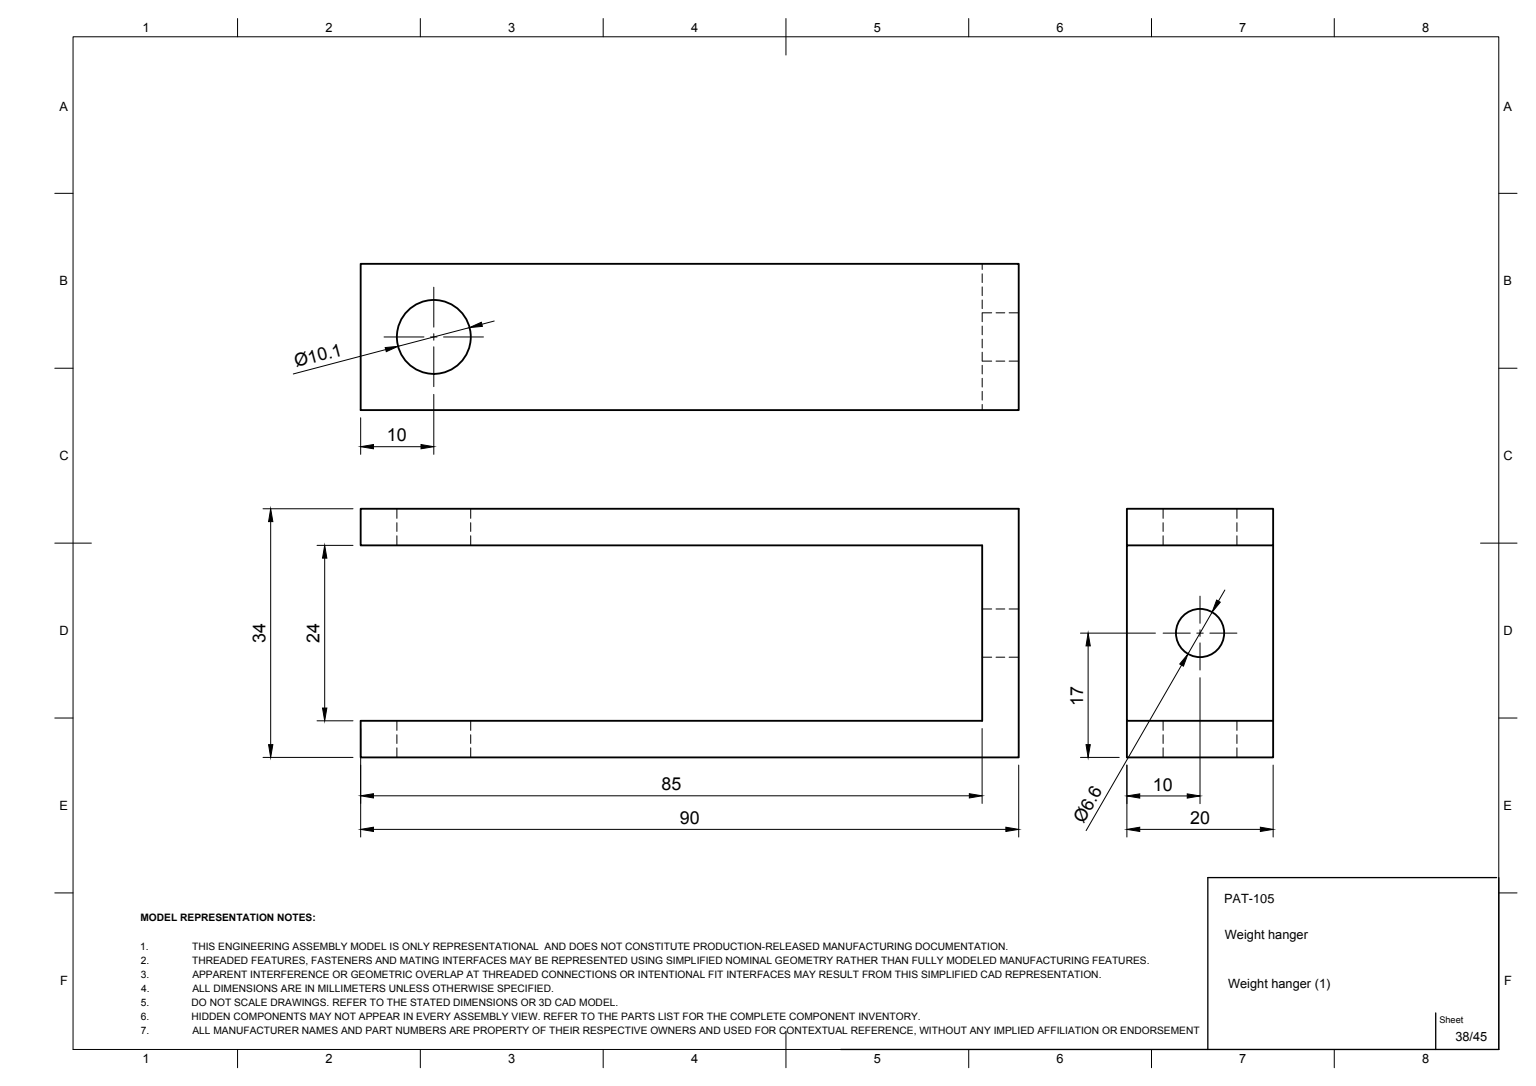
ISO-10303-21;
HEADER;
/* Generated by software containing ST-Developer
 * from STEP Tools, Inc. (www.steptools.com) 
 */

FILE_DESCRIPTION(
/* description */ ('Torque wrench calibration arm'),
/* implementation_level */ '2;1');

FILE_NAME(
/* name */ 'Weight hanger.step',
/* time_stamp */ '2026-10-28T03:24:52-07:00',
/* author */ (''),
/* organization */ (''),
/* preprocessor_version */ 'ST-DEVELOPER v20.2',
/* originating_system */ 'Autodesk Translation Framework v15.17.0.0',
/* authorisation */ '');

FILE_SCHEMA (('AUTOMOTIVE_DESIGN { 1 0 10303 214 3 1 1 }'));
ENDSEC;

DATA;
#10=MECHANICAL_DESIGN_GEOMETRIC_PRESENTATION_REPRESENTATION('',(#471),#12783);
#380=SHAPE_REPRESENTATION_RELATIONSHIP('SRR','None',#12965,#417);
#417=ADVANCED_BREP_SHAPE_REPRESENTATION('',(#523),#12774);
#471=STYLED_ITEM('',(#13198),#523);
#523=MANIFOLD_SOLID_BREP('Body1',#6542);
#631=FACE_BOUND('',#1709,.T.);
#632=FACE_BOUND('',#1712,.T.);
#633=FACE_BOUND('',#1714,.T.);
#634=FACE_BOUND('',#1716,.T.);
#635=FACE_BOUND('',#1719,.T.);
#636=FACE_BOUND('',#1723,.T.);
#838=PLANE('',#7695);
#839=PLANE('',#7696);
#840=PLANE('',#7697);
#841=PLANE('',#7698);
#842=PLANE('',#7699);
#843=PLANE('',#7700);
#844=PLANE('',#7701);
#845=PLANE('',#7702);
#846=PLANE('',#7703);
#847=PLANE('',#7704);
#1210=FACE_OUTER_BOUND('',#1705,.T.);
#1211=FACE_OUTER_BOUND('',#1706,.T.);
#1212=FACE_OUTER_BOUND('',#1707,.T.);
#1213=FACE_OUTER_BOUND('',#1708,.T.);
#1214=FACE_OUTER_BOUND('',#1710,.T.);
#1215=FACE_OUTER_BOUND('',#1711,.T.);
#1216=FACE_OUTER_BOUND('',#1713,.T.);
#1217=FACE_OUTER_BOUND('',#1715,.T.);
#1218=FACE_OUTER_BOUND('',#1717,.T.);
#1219=FACE_OUTER_BOUND('',#1718,.T.);
#1220=FACE_OUTER_BOUND('',#1720,.T.);
#1221=FACE_OUTER_BOUND('',#1721,.T.);
#1222=FACE_OUTER_BOUND('',#1722,.T.);
#1705=EDGE_LOOP('',(#5771,#5772,#5773,#5774));
#1706=EDGE_LOOP('',(#5775,#5776,#5777,#5778));
#1707=EDGE_LOOP('',(#5779,#5780,#5781,#5782));
#1708=EDGE_LOOP('',(#5783,#5784,#5785,#5786));
#1709=EDGE_LOOP('',(#5787));
#1710=EDGE_LOOP('',(#5788,#5789,#5790,#5791));
#1711=EDGE_LOOP('',(#5792,#5793,#5794,#5795));
#1712=EDGE_LOOP('',(#5796));
#1713=EDGE_LOOP('',(#5797,#5798,#5799,#5800));
#1714=EDGE_LOOP('',(#5801));
#1715=EDGE_LOOP('',(#5802,#5803,#5804,#5805));
#1716=EDGE_LOOP('',(#5806));
#1717=EDGE_LOOP('',(#5807,#5808,#5809,#5810,#5811,#5812,#5813,#5814));
#1718=EDGE_LOOP('',(#5815,#5816,#5817,#5818));
#1719=EDGE_LOOP('',(#5819));
#1720=EDGE_LOOP('',(#5820,#5821,#5822,#5823,#5824,#5825,#5826,#5827));
#1721=EDGE_LOOP('',(#5828,#5829,#5830,#5831));
#1722=EDGE_LOOP('',(#5832,#5833,#5834,#5835));
#1723=EDGE_LOOP('',(#5836));
#2136=LINE('',#12440,#2551);
#2137=LINE('',#12446,#2552);
#2138=LINE('',#12452,#2553);
#2139=LINE('',#12457,#2554);
#2140=LINE('',#12459,#2555);
#2141=LINE('',#12461,#2556);
#2142=LINE('',#12462,#2557);
#2143=LINE('',#12466,#2558);
#2144=LINE('',#12468,#2559);
#2145=LINE('',#12470,#2560);
#2146=LINE('',#12471,#2561);
#2147=LINE('',#12474,#2562);
#2148=LINE('',#12476,#2563);
#2149=LINE('',#12477,#2564);
#2150=LINE('',#12479,#2565);
#2151=LINE('',#12480,#2566);
#2152=LINE('',#12483,#2567);
#2153=LINE('',#12485,#2568);
#2154=LINE('',#12486,#2569);
#2155=LINE('',#12490,#2570);
#2156=LINE('',#12491,#2571);
#2157=LINE('',#12492,#2572);
#2158=LINE('',#12495,#2573);
#2159=LINE('',#12496,#2574);
#2160=LINE('',#12499,#2575);
#2161=LINE('',#12500,#2576);
#2162=LINE('',#12502,#2577);
#2551=VECTOR('',#9616,0.329999999999998);
#2552=VECTOR('',#9623,0.505000000000003);
#2553=VECTOR('',#9630,0.505000000000003);
#2554=VECTOR('',#9635,1.);
#2555=VECTOR('',#9636,1.);
#2556=VECTOR('',#9637,1.);
#2557=VECTOR('',#9638,1.);
#2558=VECTOR('',#9641,1.);
#2559=VECTOR('',#9642,1.);
#2560=VECTOR('',#9643,1.);
#2561=VECTOR('',#9644,1.);
#2562=VECTOR('',#9647,1.);
#2563=VECTOR('',#9648,1.);
#2564=VECTOR('',#9649,1.);
#2565=VECTOR('',#9652,1.);
#2566=VECTOR('',#9653,1.);
#2567=VECTOR('',#9656,1.);
#2568=VECTOR('',#9657,1.);
#2569=VECTOR('',#9658,1.);
#2570=VECTOR('',#9661,1.);
#2571=VECTOR('',#9662,1.);
#2572=VECTOR('',#9663,1.);
#2573=VECTOR('',#9666,1.);
#2574=VECTOR('',#9667,1.);
#2575=VECTOR('',#9670,1.);
#2576=VECTOR('',#9671,1.);
#2577=VECTOR('',#9674,1.);
#2928=CIRCLE('',#7687,0.329999999999998);
#2929=CIRCLE('',#7688,0.329999999999998);
#2930=CIRCLE('',#7690,0.505000000000003);
#2931=CIRCLE('',#7691,0.505000000000003);
#2932=CIRCLE('',#7693,0.505000000000003);
#2933=CIRCLE('',#7694,0.505000000000003);
#3462=VERTEX_POINT('',#12437);
#3463=VERTEX_POINT('',#12439);
#3464=VERTEX_POINT('',#12443);
#3465=VERTEX_POINT('',#12445);
#3466=VERTEX_POINT('',#12449);
#3467=VERTEX_POINT('',#12451);
#3468=VERTEX_POINT('',#12455);
#3469=VERTEX_POINT('',#12456);
#3470=VERTEX_POINT('',#12458);
#3471=VERTEX_POINT('',#12460);
#3472=VERTEX_POINT('',#12464);
#3473=VERTEX_POINT('',#12465);
#3474=VERTEX_POINT('',#12467);
#3475=VERTEX_POINT('',#12469);
#3476=VERTEX_POINT('',#12473);
#3477=VERTEX_POINT('',#12475);
#3478=VERTEX_POINT('',#12482);
#3479=VERTEX_POINT('',#12484);
#3480=VERTEX_POINT('',#12488);
#3481=VERTEX_POINT('',#12489);
#3482=VERTEX_POINT('',#12494);
#3483=VERTEX_POINT('',#12498);
#4243=EDGE_CURVE('',#3462,#3462,#2928,.T.);
#4244=EDGE_CURVE('',#3462,#3463,#2136,.T.);
#4245=EDGE_CURVE('',#3463,#3463,#2929,.T.);
#4246=EDGE_CURVE('',#3464,#3464,#2930,.T.);
#4247=EDGE_CURVE('',#3464,#3465,#2137,.T.);
#4248=EDGE_CURVE('',#3465,#3465,#2931,.T.);
#4249=EDGE_CURVE('',#3466,#3466,#2932,.T.);
#4250=EDGE_CURVE('',#3466,#3467,#2138,.T.);
#4251=EDGE_CURVE('',#3467,#3467,#2933,.T.);
#4252=EDGE_CURVE('',#3468,#3469,#2139,.T.);
#4253=EDGE_CURVE('',#3468,#3470,#2140,.T.);
#4254=EDGE_CURVE('',#3471,#3470,#2141,.T.);
#4255=EDGE_CURVE('',#3469,#3471,#2142,.T.);
#4256=EDGE_CURVE('',#3472,#3473,#2143,.T.);
#4257=EDGE_CURVE('',#3472,#3474,#2144,.T.);
#4258=EDGE_CURVE('',#3475,#3474,#2145,.T.);
#4259=EDGE_CURVE('',#3473,#3475,#2146,.T.);
#4260=EDGE_CURVE('',#3474,#3476,#2147,.T.);
#4261=EDGE_CURVE('',#3476,#3477,#2148,.T.);
#4262=EDGE_CURVE('',#3477,#3475,#2149,.T.);
#4263=EDGE_CURVE('',#3470,#3472,#2150,.T.);
#4264=EDGE_CURVE('',#3473,#3471,#2151,.T.);
#4265=EDGE_CURVE('',#3469,#3478,#2152,.T.);
#4266=EDGE_CURVE('',#3478,#3479,#2153,.T.);
#4267=EDGE_CURVE('',#3479,#3468,#2154,.T.);
#4268=EDGE_CURVE('',#3480,#3481,#2155,.T.);
#4269=EDGE_CURVE('',#3480,#3478,#2156,.T.);
#4270=EDGE_CURVE('',#3481,#3477,#2157,.T.);
#4271=EDGE_CURVE('',#3481,#3482,#2158,.T.);
#4272=EDGE_CURVE('',#3482,#3476,#2159,.T.);
#4273=EDGE_CURVE('',#3482,#3483,#2160,.T.);
#4274=EDGE_CURVE('',#3483,#3479,#2161,.T.);
#4275=EDGE_CURVE('',#3483,#3480,#2162,.T.);
#5771=ORIENTED_EDGE('',*,*,#4243,.F.);
#5772=ORIENTED_EDGE('',*,*,#4244,.T.);
#5773=ORIENTED_EDGE('',*,*,#4245,.F.);
#5774=ORIENTED_EDGE('',*,*,#4244,.F.);
#5775=ORIENTED_EDGE('',*,*,#4246,.F.);
#5776=ORIENTED_EDGE('',*,*,#4247,.T.);
#5777=ORIENTED_EDGE('',*,*,#4248,.F.);
#5778=ORIENTED_EDGE('',*,*,#4247,.F.);
#5779=ORIENTED_EDGE('',*,*,#4249,.F.);
#5780=ORIENTED_EDGE('',*,*,#4250,.T.);
#5781=ORIENTED_EDGE('',*,*,#4251,.F.);
#5782=ORIENTED_EDGE('',*,*,#4250,.F.);
#5783=ORIENTED_EDGE('',*,*,#4252,.F.);
#5784=ORIENTED_EDGE('',*,*,#4253,.T.);
#5785=ORIENTED_EDGE('',*,*,#4254,.F.);
#5786=ORIENTED_EDGE('',*,*,#4255,.F.);
#5787=ORIENTED_EDGE('',*,*,#4245,.T.);
#5788=ORIENTED_EDGE('',*,*,#4256,.F.);
#5789=ORIENTED_EDGE('',*,*,#4257,.T.);
#5790=ORIENTED_EDGE('',*,*,#4258,.F.);
#5791=ORIENTED_EDGE('',*,*,#4259,.F.);
#5792=ORIENTED_EDGE('',*,*,#4258,.T.);
#5793=ORIENTED_EDGE('',*,*,#4260,.T.);
#5794=ORIENTED_EDGE('',*,*,#4261,.T.);
#5795=ORIENTED_EDGE('',*,*,#4262,.T.);
#5796=ORIENTED_EDGE('',*,*,#4251,.T.);
#5797=ORIENTED_EDGE('',*,*,#4254,.T.);
#5798=ORIENTED_EDGE('',*,*,#4263,.T.);
#5799=ORIENTED_EDGE('',*,*,#4256,.T.);
#5800=ORIENTED_EDGE('',*,*,#4264,.T.);
#5801=ORIENTED_EDGE('',*,*,#4249,.T.);
#5802=ORIENTED_EDGE('',*,*,#4252,.T.);
#5803=ORIENTED_EDGE('',*,*,#4265,.T.);
#5804=ORIENTED_EDGE('',*,*,#4266,.T.);
#5805=ORIENTED_EDGE('',*,*,#4267,.T.);
#5806=ORIENTED_EDGE('',*,*,#4248,.T.);
#5807=ORIENTED_EDGE('',*,*,#4268,.F.);
#5808=ORIENTED_EDGE('',*,*,#4269,.T.);
#5809=ORIENTED_EDGE('',*,*,#4265,.F.);
#5810=ORIENTED_EDGE('',*,*,#4255,.T.);
#5811=ORIENTED_EDGE('',*,*,#4264,.F.);
#5812=ORIENTED_EDGE('',*,*,#4259,.T.);
#5813=ORIENTED_EDGE('',*,*,#4262,.F.);
#5814=ORIENTED_EDGE('',*,*,#4270,.F.);
#5815=ORIENTED_EDGE('',*,*,#4271,.F.);
#5816=ORIENTED_EDGE('',*,*,#4270,.T.);
#5817=ORIENTED_EDGE('',*,*,#4261,.F.);
#5818=ORIENTED_EDGE('',*,*,#4272,.F.);
#5819=ORIENTED_EDGE('',*,*,#4243,.T.);
#5820=ORIENTED_EDGE('',*,*,#4273,.F.);
#5821=ORIENTED_EDGE('',*,*,#4272,.T.);
#5822=ORIENTED_EDGE('',*,*,#4260,.F.);
#5823=ORIENTED_EDGE('',*,*,#4257,.F.);
#5824=ORIENTED_EDGE('',*,*,#4263,.F.);
#5825=ORIENTED_EDGE('',*,*,#4253,.F.);
#5826=ORIENTED_EDGE('',*,*,#4267,.F.);
#5827=ORIENTED_EDGE('',*,*,#4274,.F.);
#5828=ORIENTED_EDGE('',*,*,#4275,.F.);
#5829=ORIENTED_EDGE('',*,*,#4274,.T.);
#5830=ORIENTED_EDGE('',*,*,#4266,.F.);
#5831=ORIENTED_EDGE('',*,*,#4269,.F.);
#5832=ORIENTED_EDGE('',*,*,#4275,.T.);
#5833=ORIENTED_EDGE('',*,*,#4268,.T.);
#5834=ORIENTED_EDGE('',*,*,#4271,.T.);
#5835=ORIENTED_EDGE('',*,*,#4273,.T.);
#5836=ORIENTED_EDGE('',*,*,#4246,.T.);
#6080=CYLINDRICAL_SURFACE('',#7686,0.329999999999998);
#6081=CYLINDRICAL_SURFACE('',#7689,0.505000000000003);
#6082=CYLINDRICAL_SURFACE('',#7692,0.505000000000003);
#6435=ADVANCED_FACE('',(#1210),#6080,.F.);
#6436=ADVANCED_FACE('',(#1211),#6081,.F.);
#6437=ADVANCED_FACE('',(#1212),#6082,.F.);
#6438=ADVANCED_FACE('',(#1213,#631),#838,.T.);
#6439=ADVANCED_FACE('',(#1214),#839,.T.);
#6440=ADVANCED_FACE('',(#1215,#632),#840,.T.);
#6441=ADVANCED_FACE('',(#1216,#633),#841,.F.);
#6442=ADVANCED_FACE('',(#1217,#634),#842,.T.);
#6443=ADVANCED_FACE('',(#1218),#843,.T.);
#6444=ADVANCED_FACE('',(#1219,#635),#844,.T.);
#6445=ADVANCED_FACE('',(#1220),#845,.T.);
#6446=ADVANCED_FACE('',(#1221),#846,.T.);
#6447=ADVANCED_FACE('',(#1222,#636),#847,.F.);
#6542=CLOSED_SHELL('',(#6435,#6436,#6437,#6438,#6439,#6440,#6441,#6442,
#6443,#6444,#6445,#6446,#6447));
#7685=AXIS2_PLACEMENT_3D('',#12435,#9610,#9611);
#7686=AXIS2_PLACEMENT_3D('',#12436,#9612,#9613);
#7687=AXIS2_PLACEMENT_3D('',#12438,#9614,#9615);
#7688=AXIS2_PLACEMENT_3D('',#12441,#9617,#9618);
#7689=AXIS2_PLACEMENT_3D('',#12442,#9619,#9620);
#7690=AXIS2_PLACEMENT_3D('',#12444,#9621,#9622);
#7691=AXIS2_PLACEMENT_3D('',#12447,#9624,#9625);
#7692=AXIS2_PLACEMENT_3D('',#12448,#9626,#9627);
#7693=AXIS2_PLACEMENT_3D('',#12450,#9628,#9629);
#7694=AXIS2_PLACEMENT_3D('',#12453,#9631,#9632);
#7695=AXIS2_PLACEMENT_3D('',#12454,#9633,#9634);
#7696=AXIS2_PLACEMENT_3D('',#12463,#9639,#9640);
#7697=AXIS2_PLACEMENT_3D('',#12472,#9645,#9646);
#7698=AXIS2_PLACEMENT_3D('',#12478,#9650,#9651);
#7699=AXIS2_PLACEMENT_3D('',#12481,#9654,#9655);
#7700=AXIS2_PLACEMENT_3D('',#12487,#9659,#9660);
#7701=AXIS2_PLACEMENT_3D('',#12493,#9664,#9665);
#7702=AXIS2_PLACEMENT_3D('',#12497,#9668,#9669);
#7703=AXIS2_PLACEMENT_3D('',#12501,#9672,#9673);
#7704=AXIS2_PLACEMENT_3D('',#12503,#9675,#9676);
#9610=DIRECTION('axis',(0.,0.,1.));
#9611=DIRECTION('refdir',(1.,0.,0.));
#9612=DIRECTION('center_axis',(0.,0.,1.));
#9613=DIRECTION('ref_axis',(1.,0.,0.));
#9614=DIRECTION('center_axis',(0.,0.,1.));
#9615=DIRECTION('ref_axis',(1.,0.,0.));
#9616=DIRECTION('',(0.,0.,1.));
#9617=DIRECTION('center_axis',(0.,0.,-1.));
#9618=DIRECTION('ref_axis',(1.,0.,0.));
#9619=DIRECTION('center_axis',(0.,1.,0.));
#9620=DIRECTION('ref_axis',(1.,0.,0.));
#9621=DIRECTION('center_axis',(0.,1.,0.));
#9622=DIRECTION('ref_axis',(1.,0.,0.));
#9623=DIRECTION('',(0.,1.,0.));
#9624=DIRECTION('center_axis',(0.,-1.,0.));
#9625=DIRECTION('ref_axis',(1.,0.,0.));
#9626=DIRECTION('center_axis',(0.,1.,0.));
#9627=DIRECTION('ref_axis',(1.,0.,0.));
#9628=DIRECTION('center_axis',(0.,1.,0.));
#9629=DIRECTION('ref_axis',(1.,0.,0.));
#9630=DIRECTION('',(0.,1.,0.));
#9631=DIRECTION('center_axis',(0.,-1.,0.));
#9632=DIRECTION('ref_axis',(1.,0.,0.));
#9633=DIRECTION('center_axis',(0.,0.,1.));
#9634=DIRECTION('ref_axis',(1.,0.,0.));
#9635=DIRECTION('',(-1.,0.,0.));
#9636=DIRECTION('',(0.,1.,0.));
#9637=DIRECTION('',(1.,0.,0.));
#9638=DIRECTION('',(0.,1.,0.));
#9639=DIRECTION('center_axis',(0.,0.,1.));
#9640=DIRECTION('ref_axis',(1.,0.,0.));
#9641=DIRECTION('',(-1.,0.,0.));
#9642=DIRECTION('',(0.,1.,0.));
#9643=DIRECTION('',(1.,0.,0.));
#9644=DIRECTION('',(0.,1.,0.));
#9645=DIRECTION('center_axis',(0.,1.,0.));
#9646=DIRECTION('ref_axis',(0.,0.,1.));
#9647=DIRECTION('',(0.,0.,-1.));
#9648=DIRECTION('',(-1.,0.,0.));
#9649=DIRECTION('',(0.,0.,1.));
#9650=DIRECTION('center_axis',(0.,1.,0.));
#9651=DIRECTION('ref_axis',(1.,0.,0.));
#9652=DIRECTION('',(0.,0.,1.));
#9653=DIRECTION('',(0.,0.,-1.));
#9654=DIRECTION('center_axis',(0.,1.,0.));
#9655=DIRECTION('ref_axis',(0.,0.,1.));
#9656=DIRECTION('',(0.,0.,1.));
#9657=DIRECTION('',(1.,0.,0.));
#9658=DIRECTION('',(0.,0.,-1.));
#9659=DIRECTION('center_axis',(-1.,0.,0.));
#9660=DIRECTION('ref_axis',(0.,0.,1.));
#9661=DIRECTION('',(0.,0.,-1.));
#9662=DIRECTION('',(0.,1.,0.));
#9663=DIRECTION('',(0.,1.,0.));
#9664=DIRECTION('center_axis',(0.,0.,-1.));
#9665=DIRECTION('ref_axis',(-1.,0.,0.));
#9666=DIRECTION('',(1.,0.,0.));
#9667=DIRECTION('',(0.,1.,0.));
#9668=DIRECTION('center_axis',(1.,0.,0.));
#9669=DIRECTION('ref_axis',(0.,0.,-1.));
#9670=DIRECTION('',(0.,0.,1.));
#9671=DIRECTION('',(0.,1.,0.));
#9672=DIRECTION('center_axis',(0.,0.,1.));
#9673=DIRECTION('ref_axis',(1.,0.,0.));
#9674=DIRECTION('',(-1.,0.,0.));
#9675=DIRECTION('center_axis',(0.,1.,0.));
#9676=DIRECTION('ref_axis',(1.,0.,0.));
#12435=CARTESIAN_POINT('',(0.,0.,0.));
#12436=CARTESIAN_POINT('Origin',(50.,8.5,-0.1));
#12437=CARTESIAN_POINT('',(49.67,8.5,0.));
#12438=CARTESIAN_POINT('Origin',(50.,8.5,0.));
#12439=CARTESIAN_POINT('',(49.67,8.5,0.5));
#12440=CARTESIAN_POINT('',(49.67,8.5,-0.1));
#12441=CARTESIAN_POINT('Origin',(50.,8.5,0.5));
#12442=CARTESIAN_POINT('Origin',(50.,6.7,8.));
#12443=CARTESIAN_POINT('',(49.495,6.8,8.));
#12444=CARTESIAN_POINT('Origin',(50.,6.8,8.));
#12445=CARTESIAN_POINT('',(49.495,7.3,8.));
#12446=CARTESIAN_POINT('',(49.495,6.7,8.));
#12447=CARTESIAN_POINT('Origin',(50.,7.3,8.));
#12448=CARTESIAN_POINT('Origin',(50.,6.7,8.));
#12449=CARTESIAN_POINT('',(49.495,9.7,8.));
#12450=CARTESIAN_POINT('Origin',(50.,9.7,8.));
#12451=CARTESIAN_POINT('',(49.495,10.2,8.));
#12452=CARTESIAN_POINT('',(49.495,6.7,8.));
#12453=CARTESIAN_POINT('Origin',(50.,10.2,8.));
#12454=CARTESIAN_POINT('Origin',(49.,7.3,0.5));
#12455=CARTESIAN_POINT('',(51.,7.3,0.5));
#12456=CARTESIAN_POINT('',(49.,7.3,0.5));
#12457=CARTESIAN_POINT('',(49.5,7.3,0.5));
#12458=CARTESIAN_POINT('',(51.,9.7,0.5));
#12459=CARTESIAN_POINT('',(51.,7.3,0.5));
#12460=CARTESIAN_POINT('',(49.,9.7,0.5));
#12461=CARTESIAN_POINT('',(49.5,9.7,0.5));
#12462=CARTESIAN_POINT('',(49.,7.3,0.5));
#12463=CARTESIAN_POINT('Origin',(49.,9.7,9.));
#12464=CARTESIAN_POINT('',(51.,9.7,9.));
#12465=CARTESIAN_POINT('',(49.,9.7,9.));
#12466=CARTESIAN_POINT('',(51.,9.7,9.));
#12467=CARTESIAN_POINT('',(51.,10.2,9.));
#12468=CARTESIAN_POINT('',(51.,9.7,9.));
#12469=CARTESIAN_POINT('',(49.,10.2,9.));
#12470=CARTESIAN_POINT('',(51.,10.2,9.));
#12471=CARTESIAN_POINT('',(49.,9.7,9.));
#12472=CARTESIAN_POINT('Origin',(50.,10.2,4.5));
#12473=CARTESIAN_POINT('',(51.,10.2,0.));
#12474=CARTESIAN_POINT('',(51.,10.2,0.));
#12475=CARTESIAN_POINT('',(49.,10.2,0.));
#12476=CARTESIAN_POINT('',(49.,10.2,0.));
#12477=CARTESIAN_POINT('',(49.,10.2,9.));
#12478=CARTESIAN_POINT('Origin',(50.,9.7,4.5));
#12479=CARTESIAN_POINT('',(51.,9.7,0.));
#12480=CARTESIAN_POINT('',(49.,9.7,9.));
#12481=CARTESIAN_POINT('Origin',(50.,7.3,4.5));
#12482=CARTESIAN_POINT('',(49.,7.3,9.));
#12483=CARTESIAN_POINT('',(49.,7.3,9.));
#12484=CARTESIAN_POINT('',(51.,7.3,9.));
#12485=CARTESIAN_POINT('',(51.,7.3,9.));
#12486=CARTESIAN_POINT('',(51.,7.3,0.));
#12487=CARTESIAN_POINT('Origin',(49.,6.8,0.));
#12488=CARTESIAN_POINT('',(49.,6.8,9.));
#12489=CARTESIAN_POINT('',(49.,6.8,0.));
#12490=CARTESIAN_POINT('',(49.,6.8,9.));
#12491=CARTESIAN_POINT('',(49.,6.8,9.));
#12492=CARTESIAN_POINT('',(49.,6.8,0.));
#12493=CARTESIAN_POINT('Origin',(51.,6.8,0.));
#12494=CARTESIAN_POINT('',(51.,6.8,0.));
#12495=CARTESIAN_POINT('',(49.,6.8,0.));
#12496=CARTESIAN_POINT('',(51.,6.8,0.));
#12497=CARTESIAN_POINT('Origin',(51.,6.8,9.));
#12498=CARTESIAN_POINT('',(51.,6.8,9.));
#12499=CARTESIAN_POINT('',(51.,6.8,0.));
#12500=CARTESIAN_POINT('',(51.,6.8,9.));
#12501=CARTESIAN_POINT('Origin',(49.,6.8,9.));
#12502=CARTESIAN_POINT('',(51.,6.8,9.));
#12503=CARTESIAN_POINT('Origin',(50.,6.8,4.5));
#12730=UNCERTAINTY_MEASURE_WITH_UNIT(LENGTH_MEASURE(0.001),#12784,
'DISTANCE_ACCURACY_VALUE',
'Maximum model space distance between geometric entities at asserted c
onnectivities');
#12739=UNCERTAINTY_MEASURE_WITH_UNIT(LENGTH_MEASURE(0.001),#12784,
'DISTANCE_ACCURACY_VALUE',
'Maximum model space distance between geometric entities at asserted c
onnectivities');
#12774=(
GEOMETRIC_REPRESENTATION_CONTEXT(3)
GLOBAL_UNCERTAINTY_ASSIGNED_CONTEXT((#12730))
GLOBAL_UNIT_ASSIGNED_CONTEXT((#12784,#12786,#12787))
REPRESENTATION_CONTEXT('','3D')
);
#12783=(
GEOMETRIC_REPRESENTATION_CONTEXT(3)
GLOBAL_UNCERTAINTY_ASSIGNED_CONTEXT((#12739))
GLOBAL_UNIT_ASSIGNED_CONTEXT((#12784,#12786,#12787))
REPRESENTATION_CONTEXT('','3D')
);
#12784=(
LENGTH_UNIT()
NAMED_UNIT(*)
SI_UNIT(.CENTI.,.METRE.)
);
#12786=(
NAMED_UNIT(*)
PLANE_ANGLE_UNIT()
SI_UNIT($,.RADIAN.)
);
#12787=(
NAMED_UNIT(*)
SI_UNIT($,.STERADIAN.)
SOLID_ANGLE_UNIT()
);
#12822=SHAPE_DEFINITION_REPRESENTATION(#12909,#12965);
#12909=PRODUCT_DEFINITION_SHAPE('',$,#13009);
#12965=SHAPE_REPRESENTATION('',(#7685),#12774);
#12974=PRODUCT_DEFINITION_CONTEXT('part definition',#13105,'design');
#13009=PRODUCT_DEFINITION('Weight hanger','Weight hanger',#13052,#12974);
#13052=PRODUCT_DEFINITION_FORMATION('',$,#13141);
#13105=APPLICATION_CONTEXT(
'Core Data for Automotive Mechanical Design Process');
#13106=PRODUCT_CONTEXT('part definition',#13105,'mechanical');
#13141=PRODUCT('Weight hanger','Weight hanger','Weight hanger',(#13106));
#13192=COLOUR_RGB('Light Blue',0.38,0.62,0.78);
#13193=FILL_AREA_STYLE_COLOUR('',#13192);
#13194=FILL_AREA_STYLE('',(#13193));
#13195=SURFACE_STYLE_FILL_AREA(#13194);
#13196=SURFACE_SIDE_STYLE('',(#13195));
#13197=SURFACE_STYLE_USAGE(.BOTH.,#13196);
#13198=PRESENTATION_STYLE_ASSIGNMENT((#13197));
ENDSEC;
END-ISO-10303-21;
